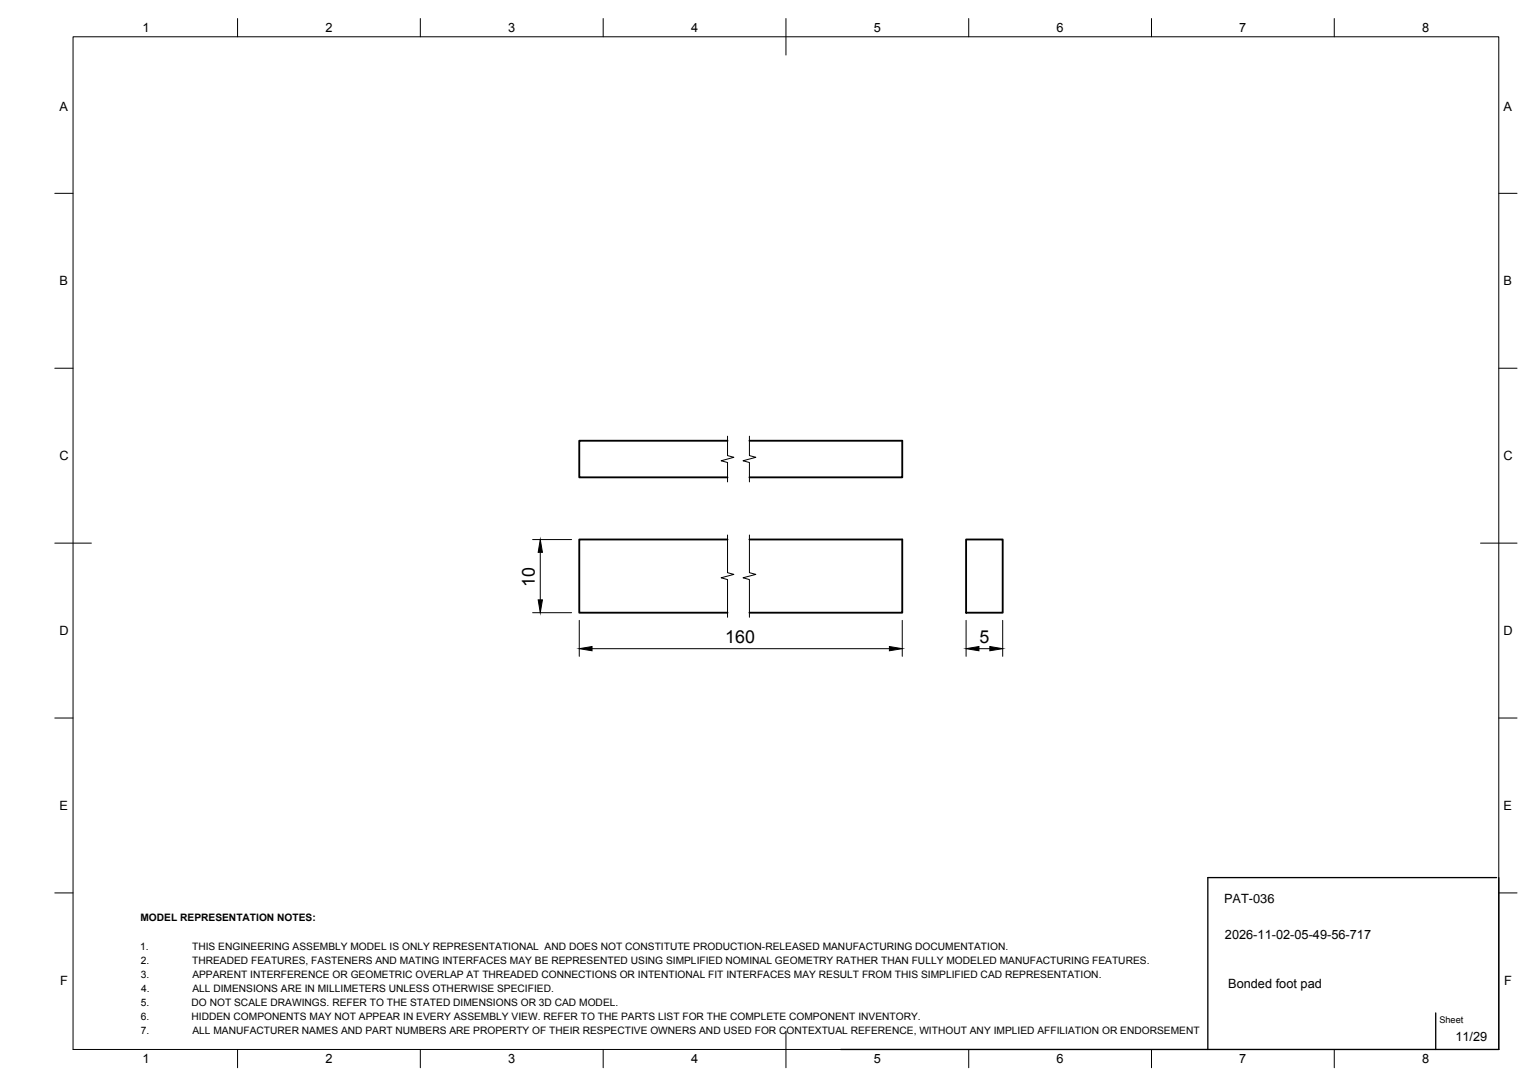
ISO-10303-21;
HEADER;
/* Generated by software containing ST-Developer
 * from STEP Tools, Inc. (www.steptools.com) 
 */

FILE_DESCRIPTION(
/* description */ ('Flange-mounted spindle'),
/* implementation_level */ '2;1');

FILE_NAME(
/* name */ 'Bonded foot pad.step',
/* time_stamp */ '2026-10-27T10:49:51-07:00',
/* author */ (''),
/* organization */ (''),
/* preprocessor_version */ 'ST-DEVELOPER v20.2',
/* originating_system */ 'Autodesk Translation Framework v15.17.0.0',
/* authorisation */ '');

FILE_SCHEMA (('AUTOMOTIVE_DESIGN { 1 0 10303 214 3 1 1 }'));
ENDSEC;

DATA;
#10=MECHANICAL_DESIGN_GEOMETRIC_PRESENTATION_REPRESENTATION('',(#344),#11764);
#290=SHAPE_REPRESENTATION_RELATIONSHIP('SRR','None',#11886,#317);
#317=ADVANCED_BREP_SHAPE_REPRESENTATION('',(#372),#11741);
#344=STYLED_ITEM('',(#12092),#372);
#372=MANIFOLD_SOLID_BREP('Body1',#6136);
#528=PLANE('',#6541);
#529=PLANE('',#6542);
#530=PLANE('',#6543);
#531=PLANE('',#6544);
#532=PLANE('',#6545);
#533=PLANE('',#6546);
#713=FACE_OUTER_BOUND('',#1084,.T.);
#714=FACE_OUTER_BOUND('',#1085,.T.);
#715=FACE_OUTER_BOUND('',#1086,.T.);
#716=FACE_OUTER_BOUND('',#1087,.T.);
#717=FACE_OUTER_BOUND('',#1088,.T.);
#718=FACE_OUTER_BOUND('',#1089,.T.);
#1084=EDGE_LOOP('',(#4167,#4168,#4169,#4170));
#1085=EDGE_LOOP('',(#4171,#4172,#4173,#4174));
#1086=EDGE_LOOP('',(#4175,#4176,#4177,#4178));
#1087=EDGE_LOOP('',(#4179,#4180,#4181,#4182));
#1088=EDGE_LOOP('',(#4183,#4184,#4185,#4186));
#1089=EDGE_LOOP('',(#4187,#4188,#4189,#4190));
#1526=LINE('',#9314,#1948);
#1527=LINE('',#9316,#1949);
#1528=LINE('',#9318,#1950);
#1529=LINE('',#9319,#1951);
#1530=LINE('',#9322,#1952);
#1531=LINE('',#9324,#1953);
#1532=LINE('',#9325,#1954);
#1533=LINE('',#9328,#1955);
#1534=LINE('',#9330,#1956);
#1535=LINE('',#9331,#1957);
#1536=LINE('',#9333,#1958);
#1537=LINE('',#9334,#1959);
#1948=VECTOR('',#7421,1.);
#1949=VECTOR('',#7422,1.);
#1950=VECTOR('',#7423,1.);
#1951=VECTOR('',#7424,1.);
#1952=VECTOR('',#7427,1.);
#1953=VECTOR('',#7428,1.);
#1954=VECTOR('',#7429,1.);
#1955=VECTOR('',#7432,1.);
#1956=VECTOR('',#7433,1.);
#1957=VECTOR('',#7434,1.);
#1958=VECTOR('',#7437,1.);
#1959=VECTOR('',#7438,1.);
#2703=VERTEX_POINT('',#9312);
#2704=VERTEX_POINT('',#9313);
#2705=VERTEX_POINT('',#9315);
#2706=VERTEX_POINT('',#9317);
#2707=VERTEX_POINT('',#9321);
#2708=VERTEX_POINT('',#9323);
#2709=VERTEX_POINT('',#9327);
#2710=VERTEX_POINT('',#9329);
#3276=EDGE_CURVE('',#2703,#2704,#1526,.T.);
#3277=EDGE_CURVE('',#2704,#2705,#1527,.T.);
#3278=EDGE_CURVE('',#2706,#2705,#1528,.T.);
#3279=EDGE_CURVE('',#2703,#2706,#1529,.T.);
#3280=EDGE_CURVE('',#2707,#2703,#1530,.T.);
#3281=EDGE_CURVE('',#2708,#2706,#1531,.T.);
#3282=EDGE_CURVE('',#2707,#2708,#1532,.T.);
#3283=EDGE_CURVE('',#2709,#2707,#1533,.T.);
#3284=EDGE_CURVE('',#2710,#2708,#1534,.T.);
#3285=EDGE_CURVE('',#2709,#2710,#1535,.T.);
#3286=EDGE_CURVE('',#2704,#2709,#1536,.T.);
#3287=EDGE_CURVE('',#2705,#2710,#1537,.T.);
#4167=ORIENTED_EDGE('',*,*,#3276,.T.);
#4168=ORIENTED_EDGE('',*,*,#3277,.T.);
#4169=ORIENTED_EDGE('',*,*,#3278,.F.);
#4170=ORIENTED_EDGE('',*,*,#3279,.F.);
#4171=ORIENTED_EDGE('',*,*,#3280,.T.);
#4172=ORIENTED_EDGE('',*,*,#3279,.T.);
#4173=ORIENTED_EDGE('',*,*,#3281,.F.);
#4174=ORIENTED_EDGE('',*,*,#3282,.F.);
#4175=ORIENTED_EDGE('',*,*,#3283,.T.);
#4176=ORIENTED_EDGE('',*,*,#3282,.T.);
#4177=ORIENTED_EDGE('',*,*,#3284,.F.);
#4178=ORIENTED_EDGE('',*,*,#3285,.F.);
#4179=ORIENTED_EDGE('',*,*,#3286,.T.);
#4180=ORIENTED_EDGE('',*,*,#3285,.T.);
#4181=ORIENTED_EDGE('',*,*,#3287,.F.);
#4182=ORIENTED_EDGE('',*,*,#3277,.F.);
#4183=ORIENTED_EDGE('',*,*,#3287,.T.);
#4184=ORIENTED_EDGE('',*,*,#3284,.T.);
#4185=ORIENTED_EDGE('',*,*,#3281,.T.);
#4186=ORIENTED_EDGE('',*,*,#3278,.T.);
#4187=ORIENTED_EDGE('',*,*,#3286,.F.);
#4188=ORIENTED_EDGE('',*,*,#3276,.F.);
#4189=ORIENTED_EDGE('',*,*,#3280,.F.);
#4190=ORIENTED_EDGE('',*,*,#3283,.F.);
#5824=ADVANCED_FACE('',(#713),#528,.T.);
#5825=ADVANCED_FACE('',(#714),#529,.T.);
#5826=ADVANCED_FACE('',(#715),#530,.T.);
#5827=ADVANCED_FACE('',(#716),#531,.T.);
#5828=ADVANCED_FACE('',(#717),#532,.T.);
#5829=ADVANCED_FACE('',(#718),#533,.F.);
#6136=CLOSED_SHELL('',(#5824,#5825,#5826,#5827,#5828,#5829));
#6540=AXIS2_PLACEMENT_3D('',#9310,#7417,#7418);
#6541=AXIS2_PLACEMENT_3D('',#9311,#7419,#7420);
#6542=AXIS2_PLACEMENT_3D('',#9320,#7425,#7426);
#6543=AXIS2_PLACEMENT_3D('',#9326,#7430,#7431);
#6544=AXIS2_PLACEMENT_3D('',#9332,#7435,#7436);
#6545=AXIS2_PLACEMENT_3D('',#9335,#7439,#7440);
#6546=AXIS2_PLACEMENT_3D('',#9336,#7441,#7442);
#7417=DIRECTION('axis',(0.,0.,1.));
#7418=DIRECTION('refdir',(1.,0.,0.));
#7419=DIRECTION('center_axis',(0.,1.,0.));
#7420=DIRECTION('ref_axis',(-1.,0.,0.));
#7421=DIRECTION('',(-1.,0.,0.));
#7422=DIRECTION('',(0.,0.,1.));
#7423=DIRECTION('',(-1.,0.,0.));
#7424=DIRECTION('',(0.,0.,1.));
#7425=DIRECTION('center_axis',(1.,0.,0.));
#7426=DIRECTION('ref_axis',(0.,1.,0.));
#7427=DIRECTION('',(0.,1.,0.));
#7428=DIRECTION('',(0.,1.,0.));
#7429=DIRECTION('',(0.,0.,1.));
#7430=DIRECTION('center_axis',(0.,-1.,0.));
#7431=DIRECTION('ref_axis',(1.,0.,0.));
#7432=DIRECTION('',(1.,0.,0.));
#7433=DIRECTION('',(1.,0.,0.));
#7434=DIRECTION('',(0.,0.,1.));
#7435=DIRECTION('center_axis',(-1.,0.,0.));
#7436=DIRECTION('ref_axis',(0.,-1.,0.));
#7437=DIRECTION('',(0.,-1.,0.));
#7438=DIRECTION('',(0.,-1.,0.));
#7439=DIRECTION('center_axis',(0.,0.,1.));
#7440=DIRECTION('ref_axis',(1.,0.,0.));
#7441=DIRECTION('center_axis',(0.,0.,1.));
#7442=DIRECTION('ref_axis',(1.,0.,0.));
#9310=CARTESIAN_POINT('',(0.,0.,0.));
#9311=CARTESIAN_POINT('Origin',(8.,-3.,-0.5));
#9312=CARTESIAN_POINT('',(8.,-3.,-0.5));
#9313=CARTESIAN_POINT('',(-8.,-3.,-0.5));
#9314=CARTESIAN_POINT('',(8.,-3.,-0.5));
#9315=CARTESIAN_POINT('',(-8.,-3.,0.));
#9316=CARTESIAN_POINT('',(-8.,-3.,-0.5));
#9317=CARTESIAN_POINT('',(8.,-3.,0.));
#9318=CARTESIAN_POINT('',(8.,-3.,0.));
#9319=CARTESIAN_POINT('',(8.,-3.,-0.5));
#9320=CARTESIAN_POINT('Origin',(8.,-4.,-0.5));
#9321=CARTESIAN_POINT('',(8.,-4.,-0.5));
#9322=CARTESIAN_POINT('',(8.,-4.,-0.5));
#9323=CARTESIAN_POINT('',(8.,-4.,0.));
#9324=CARTESIAN_POINT('',(8.,-4.,0.));
#9325=CARTESIAN_POINT('',(8.,-4.,-0.5));
#9326=CARTESIAN_POINT('Origin',(-8.,-4.,-0.5));
#9327=CARTESIAN_POINT('',(-8.,-4.,-0.5));
#9328=CARTESIAN_POINT('',(-8.,-4.,-0.5));
#9329=CARTESIAN_POINT('',(-8.,-4.,0.));
#9330=CARTESIAN_POINT('',(-8.,-4.,0.));
#9331=CARTESIAN_POINT('',(-8.,-4.,-0.5));
#9332=CARTESIAN_POINT('Origin',(-8.,-3.,-0.5));
#9333=CARTESIAN_POINT('',(-8.,-3.,-0.5));
#9334=CARTESIAN_POINT('',(-8.,-3.,0.));
#9335=CARTESIAN_POINT('Origin',(0.,-3.5,0.));
#9336=CARTESIAN_POINT('Origin',(0.,-3.5,-0.5));
#11709=UNCERTAINTY_MEASURE_WITH_UNIT(LENGTH_MEASURE(0.001),#11765,
'DISTANCE_ACCURACY_VALUE',
'Maximum model space distance between geometric entities at asserted c
onnectivities');
#11732=UNCERTAINTY_MEASURE_WITH_UNIT(LENGTH_MEASURE(0.001),#11765,
'DISTANCE_ACCURACY_VALUE',
'Maximum model space distance between geometric entities at asserted c
onnectivities');
#11741=(
GEOMETRIC_REPRESENTATION_CONTEXT(3)
GLOBAL_UNCERTAINTY_ASSIGNED_CONTEXT((#11709))
GLOBAL_UNIT_ASSIGNED_CONTEXT((#11765,#11767,#11768))
REPRESENTATION_CONTEXT('','3D')
);
#11764=(
GEOMETRIC_REPRESENTATION_CONTEXT(3)
GLOBAL_UNCERTAINTY_ASSIGNED_CONTEXT((#11732))
GLOBAL_UNIT_ASSIGNED_CONTEXT((#11765,#11767,#11768))
REPRESENTATION_CONTEXT('','3D')
);
#11765=(
LENGTH_UNIT()
NAMED_UNIT(*)
SI_UNIT(.CENTI.,.METRE.)
);
#11767=(
NAMED_UNIT(*)
PLANE_ANGLE_UNIT()
SI_UNIT($,.RADIAN.)
);
#11768=(
NAMED_UNIT(*)
SI_UNIT($,.STERADIAN.)
SOLID_ANGLE_UNIT()
);
#11777=SHAPE_DEFINITION_REPRESENTATION(#11808,#11886);
#11808=PRODUCT_DEFINITION_SHAPE('',$,#11918);
#11886=SHAPE_REPRESENTATION('',(#6540),#11741);
#11909=PRODUCT_DEFINITION_CONTEXT('part definition',#12004,'design');
#11918=PRODUCT_DEFINITION('Bonded foot pad','Bonded foot pad',#11949,#11909);
#11949=PRODUCT_DEFINITION_FORMATION('',$,#12014);
#12004=APPLICATION_CONTEXT(
'Core Data for Automotive Mechanical Design Process');
#12005=PRODUCT_CONTEXT('part definition',#12004,'mechanical');
#12014=PRODUCT('Bonded foot pad','Bonded foot pad','Bonded foot pad',(#12005));
#12086=COLOUR_RGB('Sky Blue',0.24,0.69,0.87);
#12087=FILL_AREA_STYLE_COLOUR('',#12086);
#12088=FILL_AREA_STYLE('',(#12087));
#12089=SURFACE_STYLE_FILL_AREA(#12088);
#12090=SURFACE_SIDE_STYLE('',(#12089));
#12091=SURFACE_STYLE_USAGE(.BOTH.,#12090);
#12092=PRESENTATION_STYLE_ASSIGNMENT((#12091));
ENDSEC;
END-ISO-10303-21;
